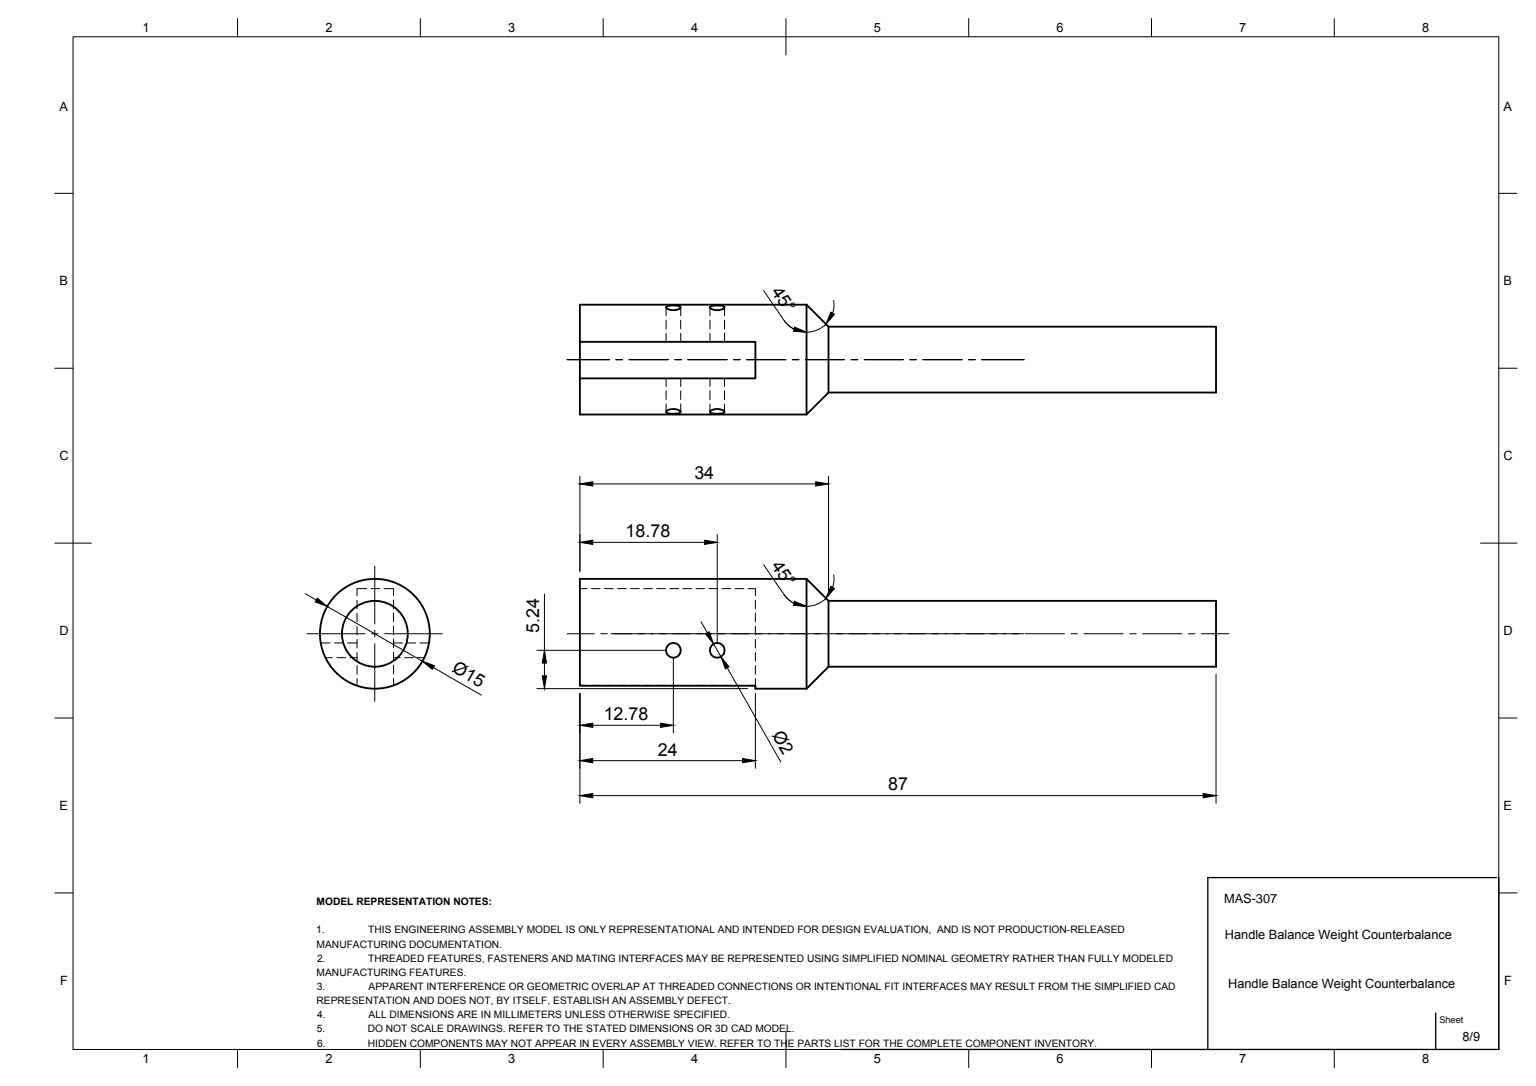
ISO-10303-21;
HEADER;
FILE_DESCRIPTION (('STEP AP214'),
    '1' );
FILE_NAME ('Handle Balance Weight Counterbalance.step',
    '2026-10-06T07:34:29',
    ( '' ),
    ( '' ),
    'SwSTEP 2.0',
    'SolidWorks 2025',
    '' );
FILE_SCHEMA (( 'AUTOMOTIVE_DESIGN' ));
ENDSEC;

DATA;
#24=CARTESIAN_POINT ( 'NONE',  ( -136.1405586187959784, 108.3975249866138597, 0.000000000000000000 ) ) ;
#39=CARTESIAN_POINT ( 'NONE',  ( -152.4086188282879277, 107.2728346664360259, 84.88378295107887084 ) ) ;
#41=CARTESIAN_POINT ( 'NONE',  ( -150.4086188282879277, 107.2728346664360259, 5.000000000000004441 ) ) ;
#42=CONICAL_SURFACE ( 'NONE', #4331, 4.499999999999950262, 0.7853981633974450594 ) ;
#130=EDGE_LOOP ( 'NONE', ( #9688, #11393, #15136, #3970 ) ) ;
#153=CARTESIAN_POINT ( 'NONE',  ( -152.0435700508773209, 108.0561044943065951, -4.829560219627783368 ) ) ;
#169=AXIS2_PLACEMENT_3D ( 'NONE', #9896, #5224, #1587 ) ;
#306=ORIENTED_EDGE ( 'NONE', *, *, #7823, .F. ) ;
#374=EDGE_LOOP ( 'NONE', ( #1367, #9906 ) ) ;
#386=CARTESIAN_POINT ( 'NONE',  ( -217.3071532141029820, 141.4846410501804712, 2.431557144026069928 ) ) ;
#394=ORIENTED_EDGE ( 'NONE', *, *, #3261, .F. ) ;
#397=CARTESIAN_POINT ( 'NONE',  ( -156.1143961258770503, 109.3137364120441077, -4.543781140870884805 ) ) ;
#425=FACE_OUTER_BOUND ( 'NONE', #2124, .T. ) ;
#429=CARTESIAN_POINT ( 'NONE',  ( -166.6414209516114795, 123.5128972754229011, 2.431557144026069928 ) ) ;
#441=AXIS2_PLACEMENT_3D ( 'NONE', #3058, #8986, #15190 ) ;
#451=DIRECTION ( 'NONE',  ( 0.000000000000000000, 0.000000000000000000, -1.000000000000000000 ) ) ;
#472=CARTESIAN_POINT ( 'NONE',  ( -142.6037198098624685, 96.81775716765160666, 0.000000000000000000 ) ) ;
#482=DIRECTION ( 'NONE',  ( -0.4873681696970814659, -0.8731965799097686221, 0.000000000000000000 ) ) ;
#505=EDGE_CURVE ( 'NONE', #2386, #1610, #1044, .T. ) ;
#514=PRESENTATION_STYLE_ASSIGNMENT (( #7896 ) ) ;
#547=CLOSED_SHELL ( 'NONE', ( #13923, #14725, #1343, #11232, #3493, #10653, #12710, #1912, #4244, #2083, #9242, #12419, #15408, #10431, #12199, #12057, #3318, #15550, #7489, #14627 ) ) ;
#588=CARTESIAN_POINT ( 'NONE',  ( -156.1569890673251280, 111.0783851182460893, -4.963902819945231748 ) ) ;
#594=CARTESIAN_POINT ( 'NONE',  ( -150.6118892440573802, 107.8916133795084846, 9.813105602333695998 ) ) ;
#621=ORIENTED_EDGE ( 'NONE', *, *, #1015, .F. ) ;
#638=DIRECTION ( 'NONE',  ( 0.000000000000000000, -0.000000000000000000, -1.000000000000000000 ) ) ;
#663=CARTESIAN_POINT ( 'NONE',  ( -155.8520457446764453, 110.8171731141052163, -4.950117075408069667 ) ) ;
#721=CARTESIAN_POINT ( 'NONE',  ( -155.6477983077465410, 110.1970436846185066, 84.88378295107887084 ) ) ;
#735=CARTESIAN_POINT ( 'NONE',  ( -152.4086188282879277, 107.2728346664360402, -4.548387523817075895 ) ) ;
#744=CARTESIAN_POINT ( 'NONE',  ( -157.1749258454821927, 111.0568882623570062, -4.859112388478813216 ) ) ;
#750=AXIS2_PLACEMENT_3D ( 'NONE', #11545, #7934, #3105 ) ;
#788=EDGE_LOOP ( 'NONE', ( #3520, #15305, #7596, #11160 ) ) ;
#858=VERTEX_POINT ( 'NONE', #6644 ) ;
#882=FACE_OUTER_BOUND ( 'NONE', #8952, .T. ) ;
#907=EDGE_LOOP ( 'NONE', ( #8993, #12549, #11670, #14820 ) ) ;
#909=CARTESIAN_POINT ( 'NONE',  ( -152.2204635237962691, 107.8706385701098185, 9.623760898223435944 ) ) ;
#981=CARTESIAN_POINT ( 'NONE',  ( -156.6477983077465410, 110.1970436846185066, 84.88378295107887084 ) ) ;
#1015=EDGE_CURVE ( 'NONE', #14712, #13022, #15364, .T. ) ;
#1025=EDGE_CURVE ( 'NONE', #9103, #13250, #7487, .T. ) ;
#1036=CARTESIAN_POINT ( 'NONE',  ( -152.2117530991619958, 106.6622082107205216, 9.223488592771907690 ) ) ;
#1044=CIRCLE ( 'NONE', #5333, 7.499999999999999112 ) ;
#1048=LINE ( 'NONE', #6988, #13883 ) ;
#1056=FACE_OUTER_BOUND ( 'NONE', #9716, .T. ) ;
#1084=CARTESIAN_POINT ( 'NONE',  ( -156.6477983077465410, 110.1970436846185066, 5.000000000000004441 ) ) ;
#1086=EDGE_LOOP ( 'NONE', ( #8415, #5150, #14250, #3362 ) ) ;
#1142=CYLINDRICAL_SURFACE ( 'NONE', #13573, 1.000000000000000888 ) ;
#1158=CARTESIAN_POINT ( 'NONE',  ( -157.6477983077465694, 110.0680497146841077, 9.367218745794341217 ) ) ;
#1159=DIRECTION ( 'NONE',  ( 0.000000000000000000, -0.000000000000000000, -1.000000000000000000 ) ) ;
#1177=ORIENTED_EDGE ( 'NONE', *, *, #7018, .T. ) ;
#1191=CARTESIAN_POINT ( 'NONE',  ( -150.9178095878665715, 108.1541761000636086, -4.963902819945232636 ) ) ;
#1200=DIRECTION ( 'NONE',  ( 0.2728218852358202384, -0.9620645606903794889, 8.659560562354905741E-17 ) ) ;
#1234=EDGE_CURVE ( 'NONE', #4804, #2746, #9270, .T. ) ;
#1285=CYLINDRICAL_SURFACE ( 'NONE', #12239, 4.499999999999950262 ) ;
#1315=CARTESIAN_POINT ( 'NONE',  ( -157.5246693090277006, 109.6988848934566647, 9.252772226370421293 ) ) ;
#1333=VERTEX_POINT ( 'NONE', #7170 ) ;
#1337=DIRECTION ( 'NONE',  ( 0.000000000000000000, 0.000000000000000000, -1.000000000000000000 ) ) ;
#1343=ADVANCED_FACE ( 'NONE', ( #11973 ), #5969, .F. ) ;
#1351=CARTESIAN_POINT ( 'NONE',  ( -157.0972765366304316, 120.0943610593438251, 0.000000000000000000 ) ) ;
#1352=CARTESIAN_POINT ( 'NONE',  ( -150.8031737844540601, 108.0798160477858261, -4.962432776364140707 ) ) ;
#1367=ORIENTED_EDGE ( 'NONE', *, *, #6082, .F. ) ;
#1404=ORIENTED_EDGE ( 'NONE', *, *, #8963, .T. ) ;
#1410=ORIENTED_EDGE ( 'NONE', *, *, #1015, .T. ) ;
#1435=CARTESIAN_POINT ( 'NONE',  ( -155.6745145678418680, 109.9335888524736049, -4.794633519332698768 ) ) ;
#1509=CARTESIAN_POINT ( 'NONE',  ( -156.1541198758405358, 111.0769426152140369, 9.827040175762295604 ) ) ;
#1557=CARTESIAN_POINT ( 'NONE',  ( -151.9345376450077367, 108.1333972819248004, 9.722517344254141491 ) ) ;
#1565=VERTEX_POINT ( 'NONE', #12048 ) ;
#1587=DIRECTION ( 'NONE',  ( -1.000000000000000000, 0.000000000000000000, 0.000000000000000000 ) ) ;
#1588=ORIENTED_EDGE ( 'NONE', *, *, #4992, .F. ) ;
#1589=CARTESIAN_POINT ( 'NONE',  ( -143.5695094297736034, 95.08739346018396077, 5.000000000000000000 ) ) ;
#1608=EDGE_CURVE ( 'NONE', #6618, #13250, #10348, .T. ) ;
#1609=DIRECTION ( 'NONE',  ( -0.4873681696970814659, -0.8731965799097686221, 0.000000000000000000 ) ) ;
#1610=VERTEX_POINT ( 'NONE', #472 ) ;
#1630=CARTESIAN_POINT ( 'NONE',  ( -156.8034031652508133, 111.1936819864191506, -4.924812526309167104 ) ) ;
#1655=AXIS2_PLACEMENT_3D ( 'NONE', #1589, #2630, #6426 ) ;
#1665=CARTESIAN_POINT ( 'NONE',  ( -155.6477983077462568, 110.3268634018094758, 9.747367390575373491 ) ) ;
#1672=EDGE_LOOP ( 'NONE', ( #11745, #12944 ) ) ;
#1778=EDGE_CURVE ( 'NONE', #858, #4152, #11112, .T. ) ;
#1784=CARTESIAN_POINT ( 'NONE',  ( -156.5388943062064584, 111.1998600659882896, -4.950241352008077023 ) ) ;
#1788=ORIENTED_EDGE ( 'NONE', *, *, #7310, .T. ) ;
#1792=SURFACE_STYLE_FILL_AREA ( #5434 ) ;
#1850=EDGE_CURVE ( 'NONE', #15505, #12940, #4802, .T. ) ;
#1867=DIRECTION ( 'NONE',  ( -0.8731965799097679559, 0.4873681696970824095, 0.000000000000000000 ) ) ;
#1884=CARTESIAN_POINT ( 'NONE',  ( -157.6477983077465694, 110.1970436846184924, 9.411501811869198875 ) ) ;
#1887=VECTOR ( 'NONE', #7298, 1000.000000000000000 ) ;
#1891=ORIENTED_EDGE ( 'NONE', *, *, #15273, .T. ) ;
#1900=CARTESIAN_POINT ( 'NONE',  ( -156.6477983077465410, 110.1970436846185066, 84.88378295107887084 ) ) ;
#1912=ADVANCED_FACE ( 'NONE', ( #10679, #15472, #4668 ), #13915, .T. ) ;
#1916=FACE_OUTER_BOUND ( 'NONE', #13980, .T. ) ;
#1925=CARTESIAN_POINT ( 'NONE',  ( -150.6072264393035027, 106.6613139020875423, -4.675203989473062371 ) ) ;
#1980=AXIS2_PLACEMENT_3D ( 'NONE', #6052, #11021, #9683 ) ;
#2014=FACE_OUTER_BOUND ( 'NONE', #8148, .T. ) ;
#2016=ORIENTED_EDGE ( 'NONE', *, *, #6082, .T. ) ;
#2066=ADVANCED_BREP_SHAPE_REPRESENTATION ( '', ( #5622, #12337 ), #10297 ) ;
#2070=DIRECTION ( 'NONE',  ( 0.000000000000000000, 0.000000000000000000, -1.000000000000000000 ) ) ;
#2083=ADVANCED_FACE ( 'NONE', ( #3484 ), #13106, .F. ) ;
#2099=DIRECTION ( 'NONE',  ( 0.000000000000000000, 0.000000000000000000, -1.000000000000000000 ) ) ;
#2104=ORIENTED_EDGE ( 'NONE', *, *, #14518, .T. ) ;
#2110=AXIS2_PLACEMENT_3D ( 'NONE', #11190, #2821, #13614 ) ;
#2124=EDGE_LOOP ( 'NONE', ( #15529, #10353, #3293, #4269 ) ) ;
#2136=DIRECTION ( 'NONE',  ( 0.000000000000000000, 0.000000000000000000, -1.000000000000000000 ) ) ;
#2159=VECTOR ( 'NONE', #14026, 1000.000000000000114 ) ;
#2242=CARTESIAN_POINT ( 'NONE',  ( -151.9050178466339105, 106.3942781637374679, -4.320071790863974748 ) ) ;
#2263=DIRECTION ( 'NONE',  ( 1.000000000000000000, 0.000000000000000000, 0.000000000000000000 ) ) ;
#2271=CARTESIAN_POINT ( 'NONE',  ( -156.3659111473432404, 109.2018789623903814, 9.312033302791148159 ) ) ;
#2284=EDGE_CURVE ( 'NONE', #8811, #8894, #6726, .T. ) ;
#2302=CARTESIAN_POINT ( 'NONE',  ( -150.6066609957502180, 106.6619251280432223, 9.538603418629666209 ) ) ;
#2303=DIRECTION ( 'NONE',  ( -0.4873681696970824651, -0.8731965799097680669, 0.000000000000000000 ) ) ;
#2323=CIRCLE ( 'NONE', #11152, 1.000000000000000888 ) ;
#2353=CARTESIAN_POINT ( 'NONE',  ( -171.0277344788851792, 115.6541280562350664, 2.431557144026069928 ) ) ;
#2386=VERTEX_POINT ( 'NONE', #3316 ) ;
#2392=DIRECTION ( 'NONE',  ( -0.8731965799097685110, 0.4873681696970817434, 0.000000000000000000 ) ) ;
#2400=CARTESIAN_POINT ( 'NONE',  ( -151.4086188282879277, 107.2728346664360259, 84.88378295107887084 ) ) ;
#2421=CIRCLE ( 'NONE', #7731, 1.000000000000000888 ) ;
#2428=CARTESIAN_POINT ( 'NONE',  ( -155.6744015425144312, 109.9339595500499343, 9.657855017614867421 ) ) ;
#2434=( NAMED_UNIT ( * ) SI_UNIT ( $, .STERADIAN. ) SOLID_ANGLE_UNIT ( ) );
#2440=DIRECTION ( 'NONE',  ( 0.8731965799097684000, -0.4873681696970815769, -0.000000000000000000 ) ) ;
#2475=DIRECTION ( 'NONE',  ( -1.000000000000000000, 0.000000000000000000, 0.000000000000000000 ) ) ;
#2525=AXIS2_PLACEMENT_3D ( 'NONE', #10287, #638, #6595 ) ;
#2536=ORIENTED_EDGE ( 'NONE', *, *, #2882, .F. ) ;
#2545=EDGE_CURVE ( 'NONE', #858, #12940, #3625, .T. ) ;
#2563=VECTOR ( 'NONE', #14577, 999.9999999999998863 ) ;
#2564=ORIENTED_EDGE ( 'NONE', *, *, #6517, .F. ) ;
#2586=DIRECTION ( 'NONE',  ( 0.000000000000000000, 0.000000000000000000, -1.000000000000000000 ) ) ;
#2590=CARTESIAN_POINT ( 'NONE',  ( -157.1465583139810178, 109.3199373332567603, 9.183240261263447834 ) ) ;
#2597=DIRECTION ( 'NONE',  ( -0.8731965799097685110, 0.4873681696970816324, -0.000000000000000000 ) ) ;
#2598=CARTESIAN_POINT ( 'NONE',  ( -168.8345777152483151, 119.5835126658289909, 2.431557144026069928 ) ) ;
#2618=CARTESIAN_POINT ( 'NONE',  ( -150.5341340129182583, 106.7708477820315665, 9.581378567423383785 ) ) ;
#2630=DIRECTION ( 'NONE',  ( -0.000000000000000000, 0.000000000000000000, 1.000000000000000000 ) ) ;
#2675=LINE ( 'NONE', #14661, #2563 ) ;
#2697=CARTESIAN_POINT ( 'NONE',  ( -152.4086188282879277, 107.2728346664360259, 0.000000000000000000 ) ) ;
#2726=FACE_OUTER_BOUND ( 'NONE', #6526, .T. ) ;
#2746=VERTEX_POINT ( 'NONE', #11432 ) ;
#2802=AXIS2_PLACEMENT_3D ( 'NONE', #14369, #9570, #2303 ) ;
#2821=DIRECTION ( 'NONE',  ( -0.8731965799097685110, 0.4873681696970816324, 0.000000000000000000 ) ) ;
#2865=CARTESIAN_POINT ( 'NONE',  ( -155.8510687235160219, 110.8158223976909369, 9.813105602333695998 ) ) ;
#2868=MECHANICAL_DESIGN_GEOMETRIC_PRESENTATION_REPRESENTATION('',(#11186),#5388);
#2882=EDGE_CURVE ( 'NONE', #11790, #2386, #5470, .T. ) ;
#2906=CARTESIAN_POINT ( 'NONE',  ( -155.6477983077465126, 110.3277548344292995, -4.884442077755424272 ) ) ;
#2933=ORIENTED_EDGE ( 'NONE', *, *, #1234, .F. ) ;
#2962=ORIENTED_EDGE ( 'NONE', *, *, #5310, .T. ) ;
#2981=FACE_BOUND ( 'NONE', #12391, .T. ) ;
#2993=DIRECTION ( 'NONE',  ( -0.000000000000000000, 0.000000000000000000, 1.000000000000000000 ) ) ;
#3058=CARTESIAN_POINT ( 'NONE',  ( -215.1139964504661464, 145.4140256597743814, 2.431557144026069928 ) ) ;
#3083=DIRECTION ( 'NONE',  ( -0.000000000000000000, 0.000000000000000000, 1.000000000000000000 ) ) ;
#3093=VERTEX_POINT ( 'NONE', #14646 ) ;
#3105=DIRECTION ( 'NONE',  ( 0.4873681696970814659, 0.8731965799097686221, 0.000000000000000000 ) ) ;
#3156=ORIENTED_EDGE ( 'NONE', *, *, #5172, .T. ) ;
#3172=ORIENTED_EDGE ( 'NONE', *, *, #5741, .T. ) ;
#3220=FACE_OUTER_BOUND ( 'NONE', #10906, .T. ) ;
#3242=EDGE_LOOP ( 'NONE', ( #3667, #6099, #3351, #12849 ) ) ;
#3261=EDGE_CURVE ( 'NONE', #14091, #858, #3588, .T. ) ;
#3293=ORIENTED_EDGE ( 'NONE', *, *, #12381, .T. ) ;
#3316=CARTESIAN_POINT ( 'NONE',  ( -135.4906327255880569, 109.5619692454514791, 2.431557144026069928 ) ) ;
#3318=ADVANCED_FACE ( 'NONE', ( #1056 ), #15561, .F. ) ;
#3332=EDGE_CURVE ( 'NONE', #13022, #11585, #2421, .T. ) ;
#3335=CARTESIAN_POINT ( 'NONE',  ( -152.4086188282879277, 107.2728346664360259, 9.411501811869209533 ) ) ;
#3351=ORIENTED_EDGE ( 'NONE', *, *, #6517, .T. ) ;
#3359=CARTESIAN_POINT ( 'NONE',  ( -150.4086188282879277, 107.2728346664360259, -4.856732557889654522 ) ) ;
#3362=ORIENTED_EDGE ( 'NONE', *, *, #8963, .F. ) ;
#3443=EDGE_CURVE ( 'NONE', #9203, #8894, #8565, .T. ) ;
#3483=CARTESIAN_POINT ( 'NONE',  ( -150.8759110177108766, 106.3887477331416989, 9.406539233868651095 ) ) ;
#3484=FACE_OUTER_BOUND ( 'NONE', #11779, .T. ) ;
#3493=ADVANCED_FACE ( 'NONE', ( #12334 ), #1285, .T. ) ;
#3506=DIRECTION ( 'NONE',  ( 0.000000000000000000, 0.000000000000000000, -1.000000000000000000 ) ) ;
#3513=ORIENTED_EDGE ( 'NONE', *, *, #4556, .F. ) ;
#3517=CARTESIAN_POINT ( 'NONE',  ( -156.6477983077465410, 110.1970436846185066, 84.88378295107887084 ) ) ;
#3520=ORIENTED_EDGE ( 'NONE', *, *, #3443, .T. ) ;
#3573=VECTOR ( 'NONE', #12281, 1000.000000000000000 ) ;
#3588=LINE ( 'NONE', #8421, #7225 ) ;
#3609=LINE ( 'NONE', #5980, #15367 ) ;
#3613=CARTESIAN_POINT ( 'NONE',  ( -157.6477983077465694, 110.1970436846184924, 9.411501811869198875 ) ) ;
#3625=LINE ( 'NONE', #13241, #13776 ) ;
#3652=CARTESIAN_POINT ( 'NONE',  ( -150.4342454288345721, 107.5345008671435920, -4.906289360893212326 ) ) ;
#3667=ORIENTED_EDGE ( 'NONE', *, *, #10642, .T. ) ;
#3669=DIRECTION ( 'NONE',  ( -0.000000000000000000, -0.000000000000000000, -1.000000000000000000 ) ) ;
#3675=AXIS2_PLACEMENT_3D ( 'NONE', #11931, #9485, #11855 ) ;
#3683=CARTESIAN_POINT ( 'NONE',  ( -150.4086188282879277, 107.2728346664360259, 0.000000000000000000 ) ) ;
#3693=SHAPE_REPRESENTATION_RELATIONSHIP ( 'NONE' , 'NONE' ,  #10258, #2066 ) ;
#3712=CARTESIAN_POINT ( 'NONE',  ( -162.5597267027908401, 124.6703825060609745, 2.431557144026069928 ) ) ;
#3730=CARTESIAN_POINT ( 'NONE',  ( -150.4086188282878425, 107.4035458162468331, -4.884442077755429601 ) ) ;
#3761=AXIS2_PLACEMENT_3D ( 'NONE', #11469, #13584, #14767 ) ;
#3787=AXIS2_PLACEMENT_3D ( 'NONE', #8092, #4432, #13990 ) ;
#3795=ORIENTED_EDGE ( 'NONE', *, *, #12897, .T. ) ;
#3813=FACE_OUTER_BOUND ( 'NONE', #788, .T. ) ;
#3823=CARTESIAN_POINT ( 'NONE',  ( -164.5262273476080850, 106.7842295329139262, 5.000000000000000000 ) ) ;
#3855=CARTESIAN_POINT ( 'NONE',  ( -150.4086188282879277, 107.2728346664360259, 84.88378295107887084 ) ) ;
#3889=FACE_BOUND ( 'NONE', #15005, .T. ) ;
#3930=CARTESIAN_POINT ( 'NONE',  ( -151.5638213263409853, 108.2696846136310711, 9.788006227097797662 ) ) ;
#3932=FACE_OUTER_BOUND ( 'NONE', #4207, .T. ) ;
#3941=PRODUCT_DEFINITION_CONTEXT ( 'detailed design', #11595, 'design' ) ;
#3954=ORIENTED_EDGE ( 'NONE', *, *, #12381, .F. ) ;
#3956=CARTESIAN_POINT ( 'NONE',  ( -157.1737171244663784, 111.0576063001072953, 9.722517344254139715 ) ) ;
#3959=PLANE ( 'NONE',  #3761 ) ;
#3966=CARTESIAN_POINT ( 'NONE',  ( -155.6477983077466263, 110.0646653313681043, -4.828669606760402466 ) ) ;
#3970=ORIENTED_EDGE ( 'NONE', *, *, #2284, .T. ) ;
#4000=CARTESIAN_POINT ( 'NONE',  ( -136.1405586187959784, 108.3975249866138597, 0.000000000000000000 ) ) ;
#4035=DIRECTION ( 'NONE',  ( -0.4873681696970824651, -0.8731965799097680669, 0.000000000000000000 ) ) ;
#4038=ORIENTED_EDGE ( 'NONE', *, *, #4337, .T. ) ;
#4078=EDGE_CURVE ( 'NONE', #5262, #6618, #8618, .T. ) ;
#4086=CARTESIAN_POINT ( 'NONE',  ( -160.1026119161506358, 114.7098309688581708, 2.431557144026069928 ) ) ;
#4107=ORIENTED_EDGE ( 'NONE', *, *, #1778, .T. ) ;
#4127=AXIS2_PLACEMENT_3D ( 'NONE', #5331, #10077, #14948 ) ;
#4148=CARTESIAN_POINT ( 'NONE',  ( -156.9354057470242765, 111.1637277590593982, -4.906715952278847936 ) ) ;
#4152=VERTEX_POINT ( 'NONE', #3712 ) ;
#4156=( NAMED_UNIT ( * ) PLANE_ANGLE_UNIT ( ) SI_UNIT ( $, .RADIAN. ) );
#4173=ORIENTED_EDGE ( 'NONE', *, *, #10294, .F. ) ;
#4207=EDGE_LOOP ( 'NONE', ( #394, #13903, #12494, #9455 ) ) ;
#4230=CARTESIAN_POINT ( 'NONE',  ( -150.9149403963819225, 108.1527335970315420, 9.827040175762299157 ) ) ;
#4233=SURFACE_SIDE_STYLE ('',( #1792 ) ) ;
#4244=ADVANCED_FACE ( 'NONE', ( #13488 ), #12536, .F. ) ;
#4263=FACE_OUTER_BOUND ( 'NONE', #130, .T. ) ;
#4269=ORIENTED_EDGE ( 'NONE', *, *, #12897, .F. ) ;
#4301=EDGE_CURVE ( 'NONE', #13018, #3093, #9168, .T. ) ;
#4305=CARTESIAN_POINT ( 'NONE',  ( -155.7763779997967504, 110.7054720168813731, -4.939346198087217310 ) ) ;
#4331=AXIS2_PLACEMENT_3D ( 'NONE', #2598, #9710, #10898 ) ;
#4337=EDGE_CURVE ( 'NONE', #13018, #5068, #13323, .T. ) ;
#4373=CARTESIAN_POINT ( 'NONE',  ( -212.9208396868292823, 149.3434102693682917, 2.431557144026069928 ) ) ;
#4391=CARTESIAN_POINT ( 'NONE',  ( -166.6414209516114795, 123.5128972754229011, 2.431557144026069928 ) ) ;
#4401=CARTESIAN_POINT ( 'NONE',  ( -155.6477983077465410, 110.1970436846185066, 5.000000000000004441 ) ) ;
#4409=DIRECTION ( 'NONE',  ( -1.000000000000000000, 0.000000000000000000, 0.000000000000000000 ) ) ;
#4432=DIRECTION ( 'NONE',  ( 0.8731965799097690661, -0.4873681696970805222, 0.000000000000000000 ) ) ;
#4435=CARTESIAN_POINT ( 'NONE',  ( -152.4086188282879277, 107.2728346664360259, 84.88378295107887084 ) ) ;
#4440=DIRECTION ( 'NONE',  ( -0.8731965799097684000, 0.4873681696970816879, 0.000000000000000000 ) ) ;
#4488=DIRECTION ( 'NONE',  ( -0.8731965799097685110, 0.4873681696970816324, -0.000000000000000000 ) ) ;
#4503=DIRECTION ( 'NONE',  ( -1.000000000000000000, 0.000000000000000000, 0.000000000000000000 ) ) ;
#4556=EDGE_CURVE ( 'NONE', #8894, #13013, #15523, .T. ) ;
#4568=CARTESIAN_POINT ( 'NONE',  ( 0.000000000000000000, 0.000000000000000000, 0.000000000000000000 ) ) ;
#4579=EDGE_LOOP ( 'NONE', ( #6858, #8658, #5081, #4990, #11443, #4173 ) ) ;
#4634=CARTESIAN_POINT ( 'NONE',  ( -157.0972765366304316, 120.0943610593438251, 0.000000000000000000 ) ) ;
#4667=CARTESIAN_POINT ( 'NONE',  ( -152.2854898295690873, 106.7746758752742124, 9.252772226370428399 ) ) ;
#4668=FACE_BOUND ( 'NONE', #15521, .T. ) ;
#4719=ORIENTED_EDGE ( 'NONE', *, *, #1608, .T. ) ;
#4728=ORIENTED_EDGE ( 'NONE', *, *, #10294, .T. ) ;
#4754=EDGE_CURVE ( 'NONE', #13295, #13013, #13398, .T. ) ;
#4800=CARTESIAN_POINT ( 'NONE',  ( -156.1150904971695752, 109.3129567513242080, 9.406539233868645766 ) ) ;
#4802=CIRCLE ( 'NONE', #14615, 7.499999999999999112 ) ;
#4804=VERTEX_POINT ( 'NONE', #9300 ) ;
#4808=CARTESIAN_POINT ( 'NONE',  ( -157.0972765366304316, 120.0943610593438251, 0.000000000000000000 ) ) ;
#4842=ORIENTED_EDGE ( 'NONE', *, *, #505, .F. ) ;
#4846=ORIENTED_EDGE ( 'NONE', *, *, #505, .T. ) ;
#4854=DIRECTION ( 'NONE',  ( 0.000000000000000000, 0.000000000000000000, -1.000000000000000000 ) ) ;
#4887=ORIENTED_EDGE ( 'NONE', *, *, #13436, .T. ) ;
#4900=ORIENTED_EDGE ( 'NONE', *, *, #5741, .F. ) ;
#4921=FACE_BOUND ( 'NONE', #1672, .T. ) ;
#4924=CARTESIAN_POINT ( 'NONE',  ( -168.8345777152483151, 119.5835126658289909, 2.431557144026069928 ) ) ;
#4950=VECTOR ( 'NONE', #12182, 999.9999999999998863 ) ;
#4952=DIRECTION ( 'NONE',  ( -0.4873681696970814659, -0.8731965799097686221, 0.000000000000000000 ) ) ;
#4982=CARTESIAN_POINT ( 'NONE',  ( -157.6477983077465694, 110.1970436846185066, 84.88378295107887084 ) ) ;
#4990=ORIENTED_EDGE ( 'NONE', *, *, #9412, .T. ) ;
#4992=EDGE_CURVE ( 'NONE', #1333, #14712, #7083, .T. ) ;
#5068=VERTEX_POINT ( 'NONE', #2697 ) ;
#5075=CARTESIAN_POINT ( 'NONE',  ( -152.2908072257909282, 107.7606257468605833, -4.720820933574416678 ) ) ;
#5081=ORIENTED_EDGE ( 'NONE', *, *, #5603, .T. ) ;
#5150=ORIENTED_EDGE ( 'NONE', *, *, #10337, .T. ) ;
#5172=EDGE_CURVE ( 'NONE', #11790, #8811, #14910, .T. ) ;
#5224=DIRECTION ( 'NONE',  ( 0.000000000000000000, 0.000000000000000000, -1.000000000000000000 ) ) ;
#5242=CIRCLE ( 'NONE', #13036, 1.000000000000000888 ) ;
#5262=VERTEX_POINT ( 'NONE', #1884 ) ;
#5289=DIRECTION ( 'NONE',  ( -0.4873681696970815769, -0.8731965799097684000, 0.000000000000000000 ) ) ;
#5299=CARTESIAN_POINT ( 'NONE',  ( -157.6233538794060962, 110.4504304370075829, 9.499964102291375667 ) ) ;
#5310=EDGE_CURVE ( 'NONE', #6421, #4804, #14826, .T. ) ;
#5315=CARTESIAN_POINT ( 'NONE',  ( -155.6477983077465410, 110.1970436846185066, -4.856732557889651858 ) ) ;
#5331=CARTESIAN_POINT ( 'NONE',  ( -151.4086188282879277, 107.2728346664360259, 0.000000000000000000 ) ) ;
#5333=AXIS2_PLACEMENT_3D ( 'NONE', #13680, #8890, #482 ) ;
#5336=DIRECTION ( 'NONE',  ( 0.8731965799097690661, -0.4873681696970805222, 0.000000000000000000 ) ) ;
#5350=DIRECTION ( 'NONE',  ( 0.9620645606903813762, 0.2728218852358138546, 0.000000000000000000 ) ) ;
#5353=( LENGTH_UNIT ( ) NAMED_UNIT ( * ) SI_UNIT ( .MILLI., .METRE. ) );
#5378=VECTOR ( 'NONE', #451, 1000.000000000000000 ) ;
#5384=CARTESIAN_POINT ( 'NONE',  ( -155.6738846654525048, 110.4594052389692962, 9.769471784547329563 ) ) ;
#5388=( GEOMETRIC_REPRESENTATION_CONTEXT ( 3 ) GLOBAL_UNCERTAINTY_ASSIGNED_CONTEXT ( ( #6756 ) ) GLOBAL_UNIT_ASSIGNED_CONTEXT ( ( #5353, #4156, #12680 ) ) REPRESENTATION_CONTEXT ( 'NONE', 'WORKASPACE' ) );
#5432=CARTESIAN_POINT ( 'NONE',  ( -150.8011781171663017, 108.0782419600532620, 9.825479475539731666 ) ) ;
#5434=FILL_AREA_STYLE ('',( #6633 ) ) ;
#5470=CIRCLE ( 'NONE', #6222, 7.499999999999999112 ) ;
#5502=CARTESIAN_POINT ( 'NONE',  ( -155.6477983077465410, 110.1970436846185066, -4.856732557889651858 ) ) ;
#5589=LINE ( 'NONE', #6703, #11121 ) ;
#5601=VECTOR ( 'NONE', #14729, 1000.000000000000000 ) ;
#5603=EDGE_CURVE ( 'NONE', #12940, #9203, #11692, .T. ) ;
#5622=MANIFOLD_SOLID_BREP ( 'Move Face2', #547 ) ;
#5629=DIRECTION ( 'NONE',  ( -0.8731965799097679559, 0.4873681696970824095, 0.000000000000000000 ) ) ;
#5634=CIRCLE ( 'NONE', #13439, 1.000000000000000888 ) ;
#5663=DIRECTION ( 'NONE',  ( 0.8731965799097684000, -0.4873681696970815769, -0.000000000000000000 ) ) ;
#5681=DIRECTION ( 'NONE',  ( 1.000000000000000000, 0.000000000000000000, 0.000000000000000000 ) ) ;
#5701=ORIENTED_EDGE ( 'NONE', *, *, #1234, .T. ) ;
#5706=CARTESIAN_POINT ( 'NONE',  ( -160.1026119161506358, 114.7098309688581708, 2.431557144026069928 ) ) ;
#5713=DIRECTION ( 'NONE',  ( 0.4873681696970831312, 0.8731965799097676229, 0.000000000000000000 ) ) ;
#5739=CARTESIAN_POINT ( 'NONE',  ( -152.3841743999474829, 107.5262214188251164, 9.499964102291382773 ) ) ;
#5741=EDGE_CURVE ( 'NONE', #11585, #13022, #11945, .T. ) ;
#5772=VECTOR ( 'NONE', #11525, 1000.000000000000000 ) ;
#5800=CARTESIAN_POINT ( 'NONE',  ( -150.8752166464184370, 106.3895273938615702, -4.543781140870890134 ) ) ;
#5808=LINE ( 'NONE', #24, #7717 ) ;
#5824=CARTESIAN_POINT ( 'NONE',  ( -136.1405586187959784, 108.3975249866138597, 0.000000000000000000 ) ) ;
#5862=CARTESIAN_POINT ( 'NONE',  ( -151.6579988274852724, 106.2951400763832766, 9.199440363476590221 ) ) ;
#5918=ORIENTED_EDGE ( 'NONE', *, *, #15246, .F. ) ;
#5949=UNCERTAINTY_MEASURE_WITH_UNIT (LENGTH_MEASURE( 1.000000000000000082E-05 ), #13157, 'distance_accuracy_value', 'NONE');
#5954=CARTESIAN_POINT ( 'NONE',  ( -152.4086188282879277, 107.2728346664360402, -4.548387523817075895 ) ) ;
#5968=DIRECTION ( 'NONE',  ( -1.000000000000000000, 0.000000000000000000, 0.000000000000000000 ) ) ;
#5969=CYLINDRICAL_SURFACE ( 'NONE', #12340, 1.000000000000000888 ) ;
#5980=CARTESIAN_POINT ( 'NONE',  ( -136.1405586187959784, 108.3975249866138597, 0.000000000000000000 ) ) ;
#5988=DIRECTION ( 'NONE',  ( 1.000000000000000000, 0.000000000000000000, 0.000000000000000000 ) ) ;
#5994=LINE ( 'NONE', #9629, #6866 ) ;
#6001=VECTOR ( 'NONE', #2597, 999.9999999999998863 ) ;
#6037=CARTESIAN_POINT ( 'NONE',  ( -151.4086188282879277, 107.2728346664360259, 5.000000000000004441 ) ) ;
#6039=DIRECTION ( 'NONE',  ( -1.000000000000000000, 0.000000000000000000, 0.000000000000000000 ) ) ;
#6052=CARTESIAN_POINT ( 'NONE',  ( -151.4086188282879277, 107.2728346664360259, 84.88378295107887084 ) ) ;
#6071=CARTESIAN_POINT ( 'NONE',  ( -157.2622295109954962, 109.3968164531734857, 9.188529295497616545 ) ) ;
#6082=EDGE_CURVE ( 'NONE', #5068, #13018, #8935, .T. ) ;
#6099=ORIENTED_EDGE ( 'NONE', *, *, #12184, .T. ) ;
#6110=CARTESIAN_POINT ( 'NONE',  ( -151.6962262675657200, 108.2395187408769033, -4.906715952278851489 ) ) ;
#6118=DIRECTION ( 'NONE',  ( 0.4873681696970831312, 0.8731965799097676229, 0.000000000000000000 ) ) ;
#6122=CARTESIAN_POINT ( 'NONE',  ( -166.2149879755189659, 118.1214081567377150, 2.431557144026069928 ) ) ;
#6222=AXIS2_PLACEMENT_3D ( 'NONE', #12051, #14257, #4952 ) ;
#6255=VERTEX_POINT ( 'NONE', #4373 ) ;
#6257=PRODUCT_CONTEXT ( 'NONE', #14795, 'mechanical' ) ;
#6264=CARTESIAN_POINT ( 'NONE',  ( -152.4086188282878993, 107.4001535559411167, -4.592095542101958472 ) ) ;
#6275=PRODUCT_DEFINITION_FORMATION_WITH_SPECIFIED_SOURCE ( 'ANY', '', #7916, .NOT_KNOWN. ) ;
#6287=ORIENTED_EDGE ( 'NONE', *, *, #7823, .T. ) ;
#6329=VERTEX_POINT ( 'NONE', #5954 ) ;
#6351=EDGE_LOOP ( 'NONE', ( #9846, #8991 ) ) ;
#6421=VERTEX_POINT ( 'NONE', #14623 ) ;
#6424=CARTESIAN_POINT ( 'NONE',  ( -156.0403575966249434, 111.0024509782357285, 9.825479475539728114 ) ) ;
#6426=DIRECTION ( 'NONE',  ( 1.000000000000000000, 0.000000000000000000, 0.000000000000000000 ) ) ;
#6437=CARTESIAN_POINT ( 'NONE',  ( -156.7587144051361179, 109.1946030148509408, -4.358407942927352785 ) ) ;
#6501=CARTESIAN_POINT ( 'NONE',  ( -157.4596430032548540, 110.7948475882922850, 9.623760898223428839 ) ) ;
#6517=EDGE_CURVE ( 'NONE', #2746, #4804, #9724, .T. ) ;
#6526=EDGE_LOOP ( 'NONE', ( #2016, #15260, #1788, #306 ) ) ;
#6546=CARTESIAN_POINT ( 'NONE',  ( -136.1405586187959784, 108.3975249866138597, 0.000000000000000000 ) ) ;
#6557=AXIS2_PLACEMENT_3D ( 'NONE', #4924, #7228, #12097 ) ;
#6595=DIRECTION ( 'NONE',  ( 1.000000000000000000, 0.000000000000000000, 0.000000000000000000 ) ) ;
#6618=VERTEX_POINT ( 'NONE', #8386 ) ;
#6624=CARTESIAN_POINT ( 'NONE',  ( -156.4041773974485920, 111.1759743691806648, -4.957866620889592291 ) ) ;
#6633=FILL_AREA_STYLE_COLOUR ( '', #6666 ) ;
#6644=CARTESIAN_POINT ( 'NONE',  ( -169.8702492482470632, 111.5724338074144413, 2.431557144026070372 ) ) ;
#6666=COLOUR_RGB ( '', 0.09019608, 0.27058824, 0.51372549) ;
#6686=ORIENTED_EDGE ( 'NONE', *, *, #14018, .T. ) ;
#6703=CARTESIAN_POINT ( 'NONE',  ( -172.2688154150754940, 113.4305367422061579, 5.000000000000000000 ) ) ;
#6712=LINE ( 'NONE', #10178, #2159 ) ;
#6726=LINE ( 'NONE', #11690, #15374 ) ;
#6756=UNCERTAINTY_MEASURE_WITH_UNIT (LENGTH_MEASURE( 1.000000000000000082E-05 ), #5353, 'distance_accuracy_value', 'NONE');
#6761=CARTESIAN_POINT ( 'NONE',  ( -151.1262866895993966, 106.2783261085441495, -4.449251264896262548 ) ) ;
#6765=DIRECTION ( 'NONE',  ( -0.000000000000000000, 0.000000000000000000, 1.000000000000000000 ) ) ;
#6844=CARTESIAN_POINT ( 'NONE',  ( -152.3062201278460748, 106.7562614988853369, -4.377525546821595448 ) ) ;
#6848=FACE_OUTER_BOUND ( 'NONE', #13888, .T. ) ;
#6849=ORIENTED_EDGE ( 'NONE', *, *, #14018, .F. ) ;
#6858=ORIENTED_EDGE ( 'NONE', *, *, #10829, .T. ) ;
#6866=VECTOR ( 'NONE', #7197, 1000.000000000000114 ) ;
#6974=AXIS2_PLACEMENT_3D ( 'NONE', #2400, #4854, #2475 ) ;
#6977=CARTESIAN_POINT ( 'NONE',  ( -152.4086188282879561, 107.1438406965016554, 9.367218745794350099 ) ) ;
#6988=CARTESIAN_POINT ( 'NONE',  ( -219.9064123261074428, 153.2423556269449421, 2.431557144026069928 ) ) ;
#7018=EDGE_CURVE ( 'NONE', #13295, #1610, #3609, .T. ) ;
#7021=EDGE_CURVE ( 'NONE', #1333, #11585, #15589, .T. ) ;
#7031=ORIENTED_EDGE ( 'NONE', *, *, #4301, .F. ) ;
#7058=AXIS2_PLACEMENT_3D ( 'NONE', #14307, #3506, #6039 ) ;
#7077=CARTESIAN_POINT ( 'NONE',  ( -152.0205871941159614, 106.4705699334293598, -4.325135862343421955 ) ) ;
#7083=B_SPLINE_CURVE_WITH_KNOTS ( 'NONE', 3,
 ( #3335, #6977, #11862, #4667, #1036, #11939, #12954, #5862, #9494, #14290, #3483, #2302, #2618, #7597, #9652, #13338 ),
 .UNSPECIFIED., .F., .F.,
 ( 4, 2, 2, 2, 2, 2, 2, 4 ),
 ( 0.000000000000000000, 0.0004036473355434109611, 0.0008072946710868219222, 0.001210942006630233046, 0.001614589342173643844, 0.002421884013260385427, 0.002825531348803770638, 0.003229178684347154982 ),
 .UNSPECIFIED. ) ;
#7154=DIRECTION ( 'NONE',  ( 0.000000000000000000, -0.000000000000000000, -1.000000000000000000 ) ) ;
#7170=CARTESIAN_POINT ( 'NONE',  ( -152.4086188282879277, 107.2728346664360259, 9.411501811869209533 ) ) ;
#7197=DIRECTION ( 'NONE',  ( 0.8731965799097684000, -0.4873681696970815769, -0.000000000000000000 ) ) ;
#7225=VECTOR ( 'NONE', #1200, 1000.000000000000114 ) ;
#7228=DIRECTION ( 'NONE',  ( -0.8731965799097685110, 0.4873681696970816324, 0.000000000000000000 ) ) ;
#7260=CARTESIAN_POINT ( 'NONE',  ( -155.6477983077462852, 110.0653742669871917, 9.691934182417337951 ) ) ;
#7293=CIRCLE ( 'NONE', #441, 4.499999999999950262 ) ;
#7298=DIRECTION ( 'NONE',  ( 0.000000000000000000, 0.000000000000000000, -1.000000000000000000 ) ) ;
#7310=EDGE_CURVE ( 'NONE', #3093, #6329, #11205, .T. ) ;
#7381=CARTESIAN_POINT ( 'NONE',  ( -152.3848650261365663, 107.5241111436813242, -4.636096941365081214 ) ) ;
#7390=DIRECTION ( 'NONE',  ( 0.8731965799097684000, -0.4873681696970816324, -0.000000000000000000 ) ) ;
#7395=DIRECTION ( 'NONE',  ( 0.8731965799097690661, -0.4873681696970805222, 0.000000000000000000 ) ) ;
#7459=CARTESIAN_POINT ( 'NONE',  ( -156.3654661690580667, 109.2025351267266586, -4.449251264896256330 ) ) ;
#7460=CARTESIAN_POINT ( 'NONE',  ( -222.0995690897442785, 149.3129710173510318, 2.431557144026069928 ) ) ;
#7487=LINE ( 'NONE', #12212, #5601 ) ;
#7488=ORIENTED_EDGE ( 'NONE', *, *, #14518, .F. ) ;
#7489=ADVANCED_FACE ( 'NONE', ( #8568 ), #15491, .F. ) ;
#7530=CARTESIAN_POINT ( 'NONE',  ( -151.9357463660236078, 108.1326792441745255, -4.859112388478815880 ) ) ;
#7570=PLANE ( 'NONE',  #14379 ) ;
#7596=ORIENTED_EDGE ( 'NONE', *, *, #5172, .F. ) ;
#7597=CARTESIAN_POINT ( 'NONE',  ( -150.4352220630557895, 107.0097505318674393, 9.657855017614867421 ) ) ;
#7621=CARTESIAN_POINT ( 'NONE',  ( -155.7734221399892363, 109.6948923088348806, -4.718200141660416236 ) ) ;
#7649=CARTESIAN_POINT ( 'NONE',  ( -157.5299867052495699, 110.6848347650430782, -4.720820933574413125 ) ) ;
#7687=CARTESIAN_POINT ( 'NONE',  ( -157.2824335677085799, 110.9804333728871057, 9.692725945294363044 ) ) ;
#7717=VECTOR ( 'NONE', #3669, 1000.000000000000000 ) ;
#7731=AXIS2_PLACEMENT_3D ( 'NONE', #6037, #7154, #10699 ) ;
#7813=ORIENTED_EDGE ( 'NONE', *, *, #3332, .T. ) ;
#7823=EDGE_CURVE ( 'NONE', #5068, #6329, #10451, .T. ) ;
#7829=ORIENTED_EDGE ( 'NONE', *, *, #4992, .T. ) ;
#7838=CARTESIAN_POINT ( 'NONE',  ( -157.6477983077465694, 110.1970436846185066, 84.88378295107887084 ) ) ;
#7847=FACE_OUTER_BOUND ( 'NONE', #3242, .T. ) ;
#7889=CARTESIAN_POINT ( 'NONE',  ( -157.4608918519057568, 110.7933268109660787, -4.760088435541717011 ) ) ;
#7896=SURFACE_STYLE_USAGE ( .BOTH. , #4233 ) ;
#7911=CARTESIAN_POINT ( 'NONE',  ( -151.4086188282879277, 107.2728346664360259, 0.000000000000000000 ) ) ;
#7916=PRODUCT ( 'Handle Balance Weight Counterbalance', 'Handle Balance Weight Counterbalance', '', ( #6257 ) ) ;
#7926=B_SPLINE_CURVE_WITH_KNOTS ( 'NONE', 3,
 ( #3613, #1158, #12135, #1315, #10805, #6071, #2590, #9537, #10964, #2271, #4800, #8448, #13228, #2428, #7260, #8518 ),
 .UNSPECIFIED., .F., .F.,
 ( 4, 2, 2, 2, 2, 2, 2, 4 ),
 ( 1.430489624538199204E-17, 0.0004036473355434303683, 0.0008072946710868464252, 0.001210942006630262536, 0.001614589342173678539, 0.002421884013260430530, 0.002825531348803793190, 0.003229178684347155416 ),
 .UNSPECIFIED. ) ;
#7934=DIRECTION ( 'NONE',  ( 0.8731965799097685110, -0.4873681696970816324, -0.000000000000000000 ) ) ;
#7946=ORIENTED_EDGE ( 'NONE', *, *, #7021, .T. ) ;
#7954=CARTESIAN_POINT ( 'NONE',  ( -150.4086188282879277, 107.1404563131855809, -4.828669606760403354 ) ) ;
#8003=CARTESIAN_POINT ( 'NONE',  ( -163.5604377276969217, 108.5145932403815721, 0.000000000000000000 ) ) ;
#8078=EDGE_LOOP ( 'NONE', ( #11298, #6849 ) ) ;
#8092=CARTESIAN_POINT ( 'NONE',  ( -166.2149879755189659, 118.1214081567377150, 2.431557144026069928 ) ) ;
#8143=DIRECTION ( 'NONE',  ( -1.000000000000000000, 0.000000000000000000, 0.000000000000000000 ) ) ;
#8147=DIRECTION ( 'NONE',  ( 0.000000000000000000, 0.000000000000000000, 1.000000000000000000 ) ) ;
#8148=EDGE_LOOP ( 'NONE', ( #12851, #13554, #2962, #5701 ) ) ;
#8196=CARTESIAN_POINT ( 'NONE',  ( -150.4353350883832832, 107.0093798342911242, -4.794633519332702321 ) ) ;
#8238=B_SPLINE_CURVE_WITH_KNOTS ( 'NONE', 3,
 ( #11430, #13544, #8752, #9943, #594, #5432, #4230, #9069, #14734, #3930, #12372, #1557, #12834, #909, #11512, #5739, #13950, #9223 ),
 .UNSPECIFIED., .F., .F.,
 ( 4, 2, 2, 2, 2, 2, 2, 2, 4 ),
 ( 0.003229178684347154982, 0.003627155556181206521, 0.004025132428015258494, 0.004423109299849310033, 0.004821086171683361572, 0.005219063043517413111, 0.005617039915351465518, 0.006015016787185517057, 0.006412993659019568596 ),
 .UNSPECIFIED. ) ;
#8280=EDGE_LOOP ( 'NONE', ( #11760, #6686, #11839, #4719 ) ) ;
#8380=EDGE_CURVE ( 'NONE', #8424, #4152, #12601, .T. ) ;
#8384=EDGE_CURVE ( 'NONE', #14712, #1333, #8238, .T. ) ;
#8386=CARTESIAN_POINT ( 'NONE',  ( -157.6477983077465694, 110.1970436846185066, 5.000000000000004441 ) ) ;
#8396=FACE_BOUND ( 'NONE', #15020, .T. ) ;
#8407=VECTOR ( 'NONE', #2070, 1000.000000000000000 ) ;
#8411=CYLINDRICAL_SURFACE ( 'NONE', #15242, 4.499999999999950262 ) ;
#8415=ORIENTED_EDGE ( 'NONE', *, *, #9015, .F. ) ;
#8419=ORIENTED_EDGE ( 'NONE', *, *, #3261, .T. ) ;
#8421=CARTESIAN_POINT ( 'NONE',  ( -171.0277344788851792, 115.6541280562350806, 2.431557144026069928 ) ) ;
#8423=AXIS2_PLACEMENT_3D ( 'NONE', #11824, #14256, #2263 ) ;
#8424=VERTEX_POINT ( 'NONE', #4391 ) ;
#8448=CARTESIAN_POINT ( 'NONE',  ( -155.8458404752088313, 109.5861341462257172, 9.538603418629666209 ) ) ;
#8450=CARTESIAN_POINT ( 'NONE',  ( -157.0972765366304316, 120.0943610593438251, 5.000000000000000000 ) ) ;
#8487=DIRECTION ( 'NONE',  ( 0.8731965799097685110, -0.4873681696970816879, -0.000000000000000000 ) ) ;
#8488=CARTESIAN_POINT ( 'NONE',  ( -151.2997148267479020, 108.2756510478057947, -4.950241352008081464 ) ) ;
#8518=CARTESIAN_POINT ( 'NONE',  ( -155.6477983077465410, 110.1970436846185066, 9.719846845941789937 ) ) ;
#8552=VECTOR ( 'NONE', #12065, 1000.000000000000000 ) ;
#8565=LINE ( 'NONE', #3823, #4950 ) ;
#8568=FACE_OUTER_BOUND ( 'NONE', #9007, .T. ) ;
#8618=LINE ( 'NONE', #4982, #8798 ) ;
#8642=CARTESIAN_POINT ( 'NONE',  ( -157.5453996073046881, 109.6804705170678034, -4.377525546821591007 ) ) ;
#8658=ORIENTED_EDGE ( 'NONE', *, *, #2545, .T. ) ;
#8682=CIRCLE ( 'NONE', #2110, 4.499999999999950262 ) ;
#8709=CARTESIAN_POINT ( 'NONE',  ( -155.6477983077465410, 110.1970436846185066, 9.719846845941789937 ) ) ;
#8752=CARTESIAN_POINT ( 'NONE',  ( -150.4347051859938915, 107.5351962207867871, 9.769471784547334892 ) ) ;
#8768=CARTESIAN_POINT ( 'NONE',  ( -139.1458939983161827, 103.0129948961282054, 2.431557144026069928 ) ) ;
#8781=CARTESIAN_POINT ( 'NONE',  ( -157.5298637219052296, 110.6847670947880573, 9.583914075210627104 ) ) ;
#8795=CARTESIAN_POINT ( 'NONE',  ( -157.2597666735746031, 109.3947789516118405, -4.325135862343416626 ) ) ;
#8798=VECTOR ( 'NONE', #1337, 1000.000000000000000 ) ;
#8811=VERTEX_POINT ( 'NONE', #10259 ) ;
#8812=AXIS2_PLACEMENT_3D ( 'NONE', #8768, #12389, #5289 ) ;
#8830=ORIENTED_EDGE ( 'NONE', *, *, #11927, .T. ) ;
#8881=CARTESIAN_POINT ( 'NONE',  ( -157.6477983077465410, 109.9391580343927473, -4.459856507254698954 ) ) ;
#8890=DIRECTION ( 'NONE',  ( -0.8731965799097685110, 0.4873681696970816324, 0.000000000000000000 ) ) ;
#8894=VERTEX_POINT ( 'NONE', #8450 ) ;
#8935=CIRCLE ( 'NONE', #4127, 1.000000000000000888 ) ;
#8944=PRODUCT_DEFINITION ( 'UNKNOWN', '', #6275, #3941 ) ;
#8952=EDGE_LOOP ( 'NONE', ( #13056, #7488, #1404, #4887 ) ) ;
#8963=EDGE_CURVE ( 'NONE', #6255, #8424, #1048, .T. ) ;
#8986=DIRECTION ( 'NONE',  ( -0.8731965799097685110, 0.4873681696970817434, 0.000000000000000000 ) ) ;
#8991=ORIENTED_EDGE ( 'NONE', *, *, #7310, .F. ) ;
#8993=ORIENTED_EDGE ( 'NONE', *, *, #11447, .T. ) ;
#8998=CARTESIAN_POINT ( 'NONE',  ( -163.7578731888787331, 108.1608566195349113, 2.431557144026070372 ) ) ;
#9007=EDGE_LOOP ( 'NONE', ( #7031, #4038, #6287, #1891 ) ) ;
#9015=EDGE_CURVE ( 'NONE', #12471, #6255, #12109, .T. ) ;
#9021=CYLINDRICAL_SURFACE ( 'NONE', #169, 1.000000000000000888 ) ;
#9069=CARTESIAN_POINT ( 'NONE',  ( -151.1638989062950031, 108.2516363225298619, 9.821053999514628430 ) ) ;
#9077=AXIS2_PLACEMENT_3D ( 'NONE', #1900, #2136, #4503 ) ;
#9103=VERTEX_POINT ( 'NONE', #11776 ) ;
#9147=CARTESIAN_POINT ( 'NONE',  ( -155.6734249082932422, 110.4587098853260585, -4.906289360893208773 ) ) ;
#9168=LINE ( 'NONE', #14038, #5772 ) ;
#9203=VERTEX_POINT ( 'NONE', #10090 ) ;
#9223=CARTESIAN_POINT ( 'NONE',  ( -152.4086188282879277, 107.2728346664360259, 9.411501811869209533 ) ) ;
#9233=DIRECTION ( 'NONE',  ( 0.000000000000000000, 0.000000000000000000, -1.000000000000000000 ) ) ;
#9242=ADVANCED_FACE ( 'NONE', ( #2981, #11196, #425 ), #7570, .F. ) ;
#9270=B_SPLINE_CURVE_WITH_KNOTS ( 'NONE', 3,
 ( #12595, #14957, #13703, #7649, #7889, #12441, #744, #4148, #1630, #1784, #6624, #588, #15034, #663, #4305, #9147, #2906, #5502 ),
 .UNSPECIFIED., .F., .F.,
 ( 4, 2, 2, 2, 2, 2, 2, 2, 4 ),
 ( 1.482148387583608474E-17, 0.0003981710496980508571, 0.0007963420993960869691, 0.001194513149094122810, 0.001592684198792158976, 0.001990855248490195142, 0.002389026298188230875, 0.002787197347886267041, 0.003185368397584303207 ),
 .UNSPECIFIED. ) ;
#9273=DIRECTION ( 'NONE',  ( -0.4873681696970816879, -0.8731965799097684000, 0.000000000000000000 ) ) ;
#9300=CARTESIAN_POINT ( 'NONE',  ( -157.6477983077465694, 110.1970436846185208, -4.548387523817069678 ) ) ;
#9324=CIRCLE ( 'NONE', #6557, 4.499999999999950262 ) ;
#9412=EDGE_CURVE ( 'NONE', #9203, #11790, #5589, .T. ) ;
#9440=CARTESIAN_POINT ( 'NONE',  ( -151.6539382783454926, 106.2940129864185366, -4.336802791931510193 ) ) ;
#9455=ORIENTED_EDGE ( 'NONE', *, *, #1778, .F. ) ;
#9485=DIRECTION ( 'NONE',  ( 0.8731965799097685110, -0.4873681696970816324, -0.000000000000000000 ) ) ;
#9494=CARTESIAN_POINT ( 'NONE',  ( -151.5230023344471704, 106.2706521918282903, 9.220837571243215791 ) ) ;
#9537=CARTESIAN_POINT ( 'NONE',  ( -156.8971783069440278, 109.2193490945657430, 9.199440363476590221 ) ) ;
#9550=PRODUCT_DEFINITION_SHAPE ( 'NONE', 'NONE',  #8944 ) ;
#9570=DIRECTION ( 'NONE',  ( -0.8731965799097680669, 0.4873681696970824651, 0.000000000000000000 ) ) ;
#9580=CARTESIAN_POINT ( 'NONE',  ( -150.6128662652177752, 107.8929640959227356, -4.950117075408072331 ) ) ;
#9629=CARTESIAN_POINT ( 'NONE',  ( -165.1793164425202178, 126.1324870151522504, 2.431557144026069928 ) ) ;
#9652=CARTESIAN_POINT ( 'NONE',  ( -150.4086188282876719, 107.1411652488047253, 9.691934182417341503 ) ) ;
#9660=DIRECTION ( 'NONE',  ( 0.8731965799097684000, -0.4873681696970816324, -0.000000000000000000 ) ) ;
#9680=CARTESIAN_POINT ( 'NONE',  ( -142.5801316981433615, 96.86001897250537240, 5.000000000000000000 ) ) ;
#9683=DIRECTION ( 'NONE',  ( -1.000000000000000000, 0.000000000000000000, 0.000000000000000000 ) ) ;
#9688=ORIENTED_EDGE ( 'NONE', *, *, #4556, .T. ) ;
#9710=DIRECTION ( 'NONE',  ( 0.8731965799097690661, -0.4873681696970805222, 0.000000000000000000 ) ) ;
#9716=EDGE_LOOP ( 'NONE', ( #621, #10955, #7946, #3172 ) ) ;
#9724=B_SPLINE_CURVE_WITH_KNOTS ( 'NONE', 3,
 ( #5315, #3966, #1435, #7621, #12414, #397, #7459, #6437, #14852, #13440, #8795, #8642, #8881, #13672 ),
 .UNSPECIFIED., .F., .F.,
 ( 4, 2, 2, 2, 2, 2, 4 ),
 ( 0.003185368397584303207, 0.003588618066394591230, 0.003991867735204879253, 0.004798367072825484789, 0.005201616741635828323, 0.005604866410446171857, 0.006411365748066773056 ),
 .UNSPECIFIED. ) ;
#9846=ORIENTED_EDGE ( 'NONE', *, *, #15273, .F. ) ;
#9896=CARTESIAN_POINT ( 'NONE',  ( -156.6477983077465410, 110.1970436846185066, 84.88378295107887084 ) ) ;
#9906=ORIENTED_EDGE ( 'NONE', *, *, #4337, .F. ) ;
#9940=DIRECTION ( 'NONE',  ( 0.000000000000000000, 0.000000000000000000, -1.000000000000000000 ) ) ;
#9943=CARTESIAN_POINT ( 'NONE',  ( -150.5358285740960014, 107.7783824288041217, 9.802099390037296800 ) ) ;
#10077=DIRECTION ( 'NONE',  ( -0.000000000000000000, 0.000000000000000000, 1.000000000000000000 ) ) ;
#10090=CARTESIAN_POINT ( 'NONE',  ( -163.5368496159778147, 108.5568550452353378, 5.000000000000000000 ) ) ;
#10132=ORIENTED_EDGE ( 'NONE', *, *, #2545, .F. ) ;
#10178=CARTESIAN_POINT ( 'NONE',  ( -172.2924035267946294, 113.3882749373523922, 0.000000000000000000 ) ) ;
#10205=CARTESIAN_POINT ( 'NONE',  ( -155.7750080535546147, 110.7025914469866308, 9.802099390037289695 ) ) ;
#10223=PLANE ( 'NONE',  #14238 ) ;
#10258=SHAPE_REPRESENTATION ( 'Handle Balance Weight Counterbalance', ( #12337 ), #10297 ) ;
#10259=CARTESIAN_POINT ( 'NONE',  ( -136.1405586187959784, 108.3975249866138739, 5.000000000000000000 ) ) ;
#10287=CARTESIAN_POINT ( 'NONE',  ( -156.6477983077465410, 110.1970436846185066, 5.000000000000004441 ) ) ;
#10294=EDGE_CURVE ( 'NONE', #4152, #2386, #5994, .T. ) ;
#10297=( GEOMETRIC_REPRESENTATION_CONTEXT ( 3 ) GLOBAL_UNCERTAINTY_ASSIGNED_CONTEXT ( ( #5949 ) ) GLOBAL_UNIT_ASSIGNED_CONTEXT ( ( #13157, #14497, #2434 ) ) REPRESENTATION_CONTEXT ( 'NONE', 'WORKASPACE' ) );
#10314=CARTESIAN_POINT ( 'NONE',  ( -168.8345777152483151, 119.5835126658289909, 2.431557144026069928 ) ) ;
#10335=CYLINDRICAL_SURFACE ( 'NONE', #10457, 1.000000000000000888 ) ;
#10337=EDGE_CURVE ( 'NONE', #12471, #14091, #2675, .T. ) ;
#10348=CIRCLE ( 'NONE', #2525, 1.000000000000000888 ) ;
#10353=ORIENTED_EDGE ( 'NONE', *, *, #4754, .T. ) ;
#10431=ADVANCED_FACE ( 'NONE', ( #3932 ), #42, .T. ) ;
#10451=LINE ( 'NONE', #4435, #8407 ) ;
#10457=AXIS2_PLACEMENT_3D ( 'NONE', #11679, #9233, #8143 ) ;
#10477=DIRECTION ( 'NONE',  ( -1.000000000000000000, 0.000000000000000000, 0.000000000000000000 ) ) ;
#10512=FACE_OUTER_BOUND ( 'NONE', #8280, .T. ) ;
#10539=B_SPLINE_CURVE_WITH_KNOTS ( 'NONE', 3,
 ( #12022, #6264, #7381, #5075, #14691, #153, #7530, #6110, #14533, #8488, #12327, #1191, #1352, #9580, #13270, #3652, #3730, #11003 ),
 .UNSPECIFIED., .F., .F.,
 ( 4, 2, 2, 2, 2, 2, 2, 2, 4 ),
 ( 1.453963218420191702E-17, 0.0003981710496980498271, 0.0007963420993960851259, 0.001194513149094120425, 0.001592684198792155724, 0.001990855248490191239, 0.002389026298188226538, 0.002787197347886261837, 0.003185368397584297136 ),
 .UNSPECIFIED. ) ;
#10642=EDGE_CURVE ( 'NONE', #6421, #1565, #2323, .T. ) ;
#10653=ADVANCED_FACE ( 'NONE', ( #6848 ), #12896, .T. ) ;
#10679=FACE_OUTER_BOUND ( 'NONE', #12027, .T. ) ;
#10699=DIRECTION ( 'NONE',  ( 1.000000000000000000, 0.000000000000000000, 0.000000000000000000 ) ) ;
#10800=DIRECTION ( 'NONE',  ( -0.4873681696970824651, -0.8731965799097680669, 0.000000000000000000 ) ) ;
#10805=CARTESIAN_POINT ( 'NONE',  ( -157.4509325786206091, 109.5864172289029881, 9.223488592771900585 ) ) ;
#10829=EDGE_CURVE ( 'NONE', #4152, #858, #10844, .T. ) ;
#10844=CIRCLE ( 'NONE', #12090, 7.499999999999999112 ) ;
#10898=DIRECTION ( 'NONE',  ( 0.4873681696970831312, 0.8731965799097676229, 0.000000000000000000 ) ) ;
#10906=EDGE_LOOP ( 'NONE', ( #7829, #1410, #7813, #12179 ) ) ;
#10955=ORIENTED_EDGE ( 'NONE', *, *, #8384, .T. ) ;
#10964=CARTESIAN_POINT ( 'NONE',  ( -156.7621818139058405, 109.1948612100107994, 9.220837571243208686 ) ) ;
#11000=ORIENTED_EDGE ( 'NONE', *, *, #10829, .F. ) ;
#11003=CARTESIAN_POINT ( 'NONE',  ( -150.4086188282879277, 107.2728346664360259, -4.856732557889654522 ) ) ;
#11005=ORIENTED_EDGE ( 'NONE', *, *, #1850, .T. ) ;
#11021=DIRECTION ( 'NONE',  ( 0.000000000000000000, 0.000000000000000000, -1.000000000000000000 ) ) ;
#11101=CYLINDRICAL_SURFACE ( 'NONE', #1980, 1.000000000000000888 ) ;
#11112=CIRCLE ( 'NONE', #3787, 7.499999999999999112 ) ;
#11121=VECTOR ( 'NONE', #5663, 1000.000000000000114 ) ;
#11152=AXIS2_PLACEMENT_3D ( 'NONE', #12665, #6765, #12822 ) ;
#11160=ORIENTED_EDGE ( 'NONE', *, *, #9412, .F. ) ;
#11186=STYLED_ITEM ( 'NONE', ( #514 ), #5622 ) ;
#11190=CARTESIAN_POINT ( 'NONE',  ( -168.8345777152483151, 119.5835126658289909, 2.431557144026069928 ) ) ;
#11196=FACE_BOUND ( 'NONE', #374, .T. ) ;
#11205=B_SPLINE_CURVE_WITH_KNOTS ( 'NONE', 3,
 ( #3359, #7954, #8196, #12974, #1925, #5800, #6761, #15414, #9440, #2242, #7077, #6844, #11884, #735 ),
 .UNSPECIFIED., .F., .F.,
 ( 4, 2, 2, 2, 2, 2, 4 ),
 ( 0.003185368397584297136, 0.003588618066394599470, 0.003991867735204901804, 0.004798367072825479585, 0.005201616741635807506, 0.005604866410446135427, 0.006411365748066763515 ),
 .UNSPECIFIED. ) ;
#11232=ADVANCED_FACE ( 'NONE', ( #3220 ), #10335, .F. ) ;
#11298=ORIENTED_EDGE ( 'NONE', *, *, #11447, .F. ) ;
#11393=ORIENTED_EDGE ( 'NONE', *, *, #4754, .F. ) ;
#11430=CARTESIAN_POINT ( 'NONE',  ( -150.4086188282879277, 107.2728346664360259, 9.719846845941791713 ) ) ;
#11432=CARTESIAN_POINT ( 'NONE',  ( -155.6477983077465410, 110.1970436846185066, -4.856732557889651858 ) ) ;
#11437=AXIS2_PLACEMENT_3D ( 'NONE', #4086, #1867, #12606 ) ;
#11438=CARTESIAN_POINT ( 'NONE',  ( -156.6477983077465410, 110.1970436846185066, 0.000000000000000000 ) ) ;
#11443=ORIENTED_EDGE ( 'NONE', *, *, #2882, .T. ) ;
#11447=EDGE_CURVE ( 'NONE', #5262, #9103, #7926, .T. ) ;
#11469=CARTESIAN_POINT ( 'NONE',  ( -136.1405586187959784, 108.3975249866138597, 0.000000000000000000 ) ) ;
#11512=CARTESIAN_POINT ( 'NONE',  ( -152.2906842424466163, 107.7605580766055766, 9.583914075210632433 ) ) ;
#11525=DIRECTION ( 'NONE',  ( 0.000000000000000000, 0.000000000000000000, -1.000000000000000000 ) ) ;
#11545=CARTESIAN_POINT ( 'NONE',  ( -168.8345777152483151, 119.5835126658289909, 2.431557144026069928 ) ) ;
#11557=LINE ( 'NONE', #721, #1887 ) ;
#11572=DIRECTION ( 'NONE',  ( 0.4873681696970831312, 0.8731965799097676229, 0.000000000000000000 ) ) ;
#11585=VERTEX_POINT ( 'NONE', #12513 ) ;
#11595=APPLICATION_CONTEXT ( 'automotive_design' ) ;
#11615=AXIS2_PLACEMENT_3D ( 'NONE', #14151, #2392, #11792 ) ;
#11670=ORIENTED_EDGE ( 'NONE', *, *, #14145, .T. ) ;
#11679=CARTESIAN_POINT ( 'NONE',  ( -151.4086188282879277, 107.2728346664360259, 84.88378295107887084 ) ) ;
#11690=CARTESIAN_POINT ( 'NONE',  ( -136.1405586187959784, 108.3975249866138597, 5.000000000000000000 ) ) ;
#11692=CIRCLE ( 'NONE', #11437, 7.499999999999999112 ) ;
#11696=B_SPLINE_CURVE_WITH_KNOTS ( 'NONE', 3,
 ( #8709, #1665, #5384, #10205, #2865, #6424, #1509, #13501, #14763, #13738, #14995, #3956, #7687, #6501, #8781, #5299, #14836, #13660 ),
 .UNSPECIFIED., .F., .F.,
 ( 4, 2, 2, 2, 2, 2, 2, 2, 4 ),
 ( 0.003229178684347155416, 0.003627155556181209124, 0.004025132428015262831, 0.004423109299849316105, 0.004821086171683369379, 0.005219063043517423520, 0.005617039915351476793, 0.006015016787185530067, 0.006412993659019584208 ),
 .UNSPECIFIED. ) ;
#11719=CARTESIAN_POINT ( 'NONE',  ( -215.1139964504661464, 145.4140256597743814, 2.431557144026069928 ) ) ;
#11745=ORIENTED_EDGE ( 'NONE', *, *, #1608, .F. ) ;
#11759=ORIENTED_EDGE ( 'NONE', *, *, #3443, .F. ) ;
#11760=ORIENTED_EDGE ( 'NONE', *, *, #1025, .F. ) ;
#11775=CYLINDRICAL_SURFACE ( 'NONE', #3675, 7.499999999999999112 ) ;
#11776=CARTESIAN_POINT ( 'NONE',  ( -155.6477983077465410, 110.1970436846185066, 9.719846845941789937 ) ) ;
#11779=EDGE_LOOP ( 'NONE', ( #3954, #3513, #11759, #14782, #14778 ) ) ;
#11790=VERTEX_POINT ( 'NONE', #9680 ) ;
#11792=DIRECTION ( 'NONE',  ( -0.4873681696970831312, -0.8731965799097676229, 0.000000000000000000 ) ) ;
#11824=CARTESIAN_POINT ( 'NONE',  ( -151.4086188282879277, 107.2728346664360259, 5.000000000000004441 ) ) ;
#11839=ORIENTED_EDGE ( 'NONE', *, *, #4078, .T. ) ;
#11854=ORIENTED_EDGE ( 'NONE', *, *, #3332, .F. ) ;
#11855=DIRECTION ( 'NONE',  ( 0.4873681696970814659, 0.8731965799097686221, 0.000000000000000000 ) ) ;
#11862=CARTESIAN_POINT ( 'NONE',  ( -152.3840324909117214, 107.0166450474691260, 9.325089004845759533 ) ) ;
#11884=CARTESIAN_POINT ( 'NONE',  ( -152.4086188282879277, 107.0149490162102808, -4.459856507254708724 ) ) ;
#11927=EDGE_CURVE ( 'NONE', #8811, #13295, #5808, .T. ) ;
#11931=CARTESIAN_POINT ( 'NONE',  ( -168.8345777152483151, 119.5835126658289909, 2.431557144026069928 ) ) ;
#11939=CARTESIAN_POINT ( 'NONE',  ( -152.0230500315369397, 106.4726074349910760, 9.188529295497623650 ) ) ;
#11945=CIRCLE ( 'NONE', #8423, 1.000000000000000888 ) ;
#11973=FACE_OUTER_BOUND ( 'NONE', #907, .T. ) ;
#12022=CARTESIAN_POINT ( 'NONE',  ( -152.4086188282879277, 107.2728346664360402, -4.548387523817075895 ) ) ;
#12027=EDGE_LOOP ( 'NONE', ( #10132, #4107, #4728, #4846, #3795, #11005 ) ) ;
#12048=CARTESIAN_POINT ( 'NONE',  ( -155.6477983077465410, 110.1970436846185066, 0.000000000000000000 ) ) ;
#12051=CARTESIAN_POINT ( 'NONE',  ( -139.1458939983161827, 103.0129948961282054, 2.431557144026069928 ) ) ;
#12057=ADVANCED_FACE ( 'NONE', ( #1916 ), #10223, .T. ) ;
#12065=DIRECTION ( 'NONE',  ( -0.000000000000000000, -0.000000000000000000, -1.000000000000000000 ) ) ;
#12090=AXIS2_PLACEMENT_3D ( 'NONE', #6122, #7395, #1609 ) ;
#12097=DIRECTION ( 'NONE',  ( -0.4873681696970831312, -0.8731965799097676229, 0.000000000000000000 ) ) ;
#12109=CIRCLE ( 'NONE', #11615, 4.499999999999950262 ) ;
#12135=CARTESIAN_POINT ( 'NONE',  ( -157.6232119703703631, 109.9408540656516067, 9.325089004845752427 ) ) ;
#12179=ORIENTED_EDGE ( 'NONE', *, *, #7021, .F. ) ;
#12182=DIRECTION ( 'NONE',  ( 0.4873681696970824651, 0.8731965799097680669, 0.000000000000000000 ) ) ;
#12184=EDGE_CURVE ( 'NONE', #1565, #2746, #11557, .T. ) ;
#12199=ADVANCED_FACE ( 'NONE', ( #882 ), #8411, .T. ) ;
#12212=CARTESIAN_POINT ( 'NONE',  ( -155.6477983077465410, 110.1970436846185066, 84.88378295107887084 ) ) ;
#12239=AXIS2_PLACEMENT_3D ( 'NONE', #7460, #7390, #6118 ) ;
#12281=DIRECTION ( 'NONE',  ( 0.000000000000000000, 0.000000000000000000, -1.000000000000000000 ) ) ;
#12285=AXIS2_PLACEMENT_3D ( 'NONE', #7911, #3083, #4409 ) ;
#12327=CARTESIAN_POINT ( 'NONE',  ( -151.1649979179899219, 108.2517653509981841, -4.957866620889593179 ) ) ;
#12334=FACE_OUTER_BOUND ( 'NONE', #1086, .T. ) ;
#12337=AXIS2_PLACEMENT_3D ( 'NONE', #4568, #8147, #5681 ) ;
#12340=AXIS2_PLACEMENT_3D ( 'NONE', #981, #15423, #10477 ) ;
#12372=CARTESIAN_POINT ( 'NONE',  ( -151.6951454547776166, 108.2398202450613098, 9.769994122432189343 ) ) ;
#12381=EDGE_CURVE ( 'NONE', #13013, #15505, #13581, .T. ) ;
#12389=DIRECTION ( 'NONE',  ( -0.8731965799097685110, 0.4873681696970816324, 0.000000000000000000 ) ) ;
#12391=EDGE_LOOP ( 'NONE', ( #15231, #13248 ) ) ;
#12393=DIRECTION ( 'NONE',  ( 0.4873681696970815769, 0.8731965799097684000, 0.000000000000000000 ) ) ;
#12414=CARTESIAN_POINT ( 'NONE',  ( -155.8464059187621444, 109.5855229202700087, -4.675203989473057931 ) ) ;
#12419=ADVANCED_FACE ( 'NONE', ( #4921, #3889, #3813 ), #13430, .F. ) ;
#12441=CARTESIAN_POINT ( 'NONE',  ( -157.2827495303359626, 110.9803135124890616, -4.829560219627786921 ) ) ;
#12471=VERTEX_POINT ( 'NONE', #386 ) ;
#12494=ORIENTED_EDGE ( 'NONE', *, *, #8380, .T. ) ;
#12513=CARTESIAN_POINT ( 'NONE',  ( -152.4086188282879277, 107.2728346664360259, 5.000000000000004441 ) ) ;
#12536=PLANE ( 'NONE',  #8812 ) ;
#12549=ORIENTED_EDGE ( 'NONE', *, *, #1025, .T. ) ;
#12595=CARTESIAN_POINT ( 'NONE',  ( -157.6477983077465694, 110.1970436846185208, -4.548387523817069678 ) ) ;
#12601=LINE ( 'NONE', #429, #13571 ) ;
#12606=DIRECTION ( 'NONE',  ( -0.4873681696970814659, -0.8731965799097686221, 0.000000000000000000 ) ) ;
#12665=CARTESIAN_POINT ( 'NONE',  ( -156.6477983077465410, 110.1970436846185066, 0.000000000000000000 ) ) ;
#12680=( NAMED_UNIT ( * ) SI_UNIT ( $, .STERADIAN. ) SOLID_ANGLE_UNIT ( ) );
#12687=DIRECTION ( 'NONE',  ( -1.000000000000000000, 0.000000000000000000, 0.000000000000000000 ) ) ;
#12710=ADVANCED_FACE ( 'NONE', ( #15533, #8396, #13095 ), #11775, .T. ) ;
#12822=DIRECTION ( 'NONE',  ( -1.000000000000000000, 0.000000000000000000, 0.000000000000000000 ) ) ;
#12834=CARTESIAN_POINT ( 'NONE',  ( -152.0432540882499666, 108.0562243547046535, 9.692725945294370149 ) ) ;
#12849=ORIENTED_EDGE ( 'NONE', *, *, #5310, .F. ) ;
#12851=ORIENTED_EDGE ( 'NONE', *, *, #12184, .F. ) ;
#12870=CYLINDRICAL_SURFACE ( 'NONE', #9077, 1.000000000000000888 ) ;
#12896=CONICAL_SURFACE ( 'NONE', #15164, 4.499999999999950262, 0.7853981633974450594 ) ;
#12897=EDGE_CURVE ( 'NONE', #1610, #15505, #6712, .T. ) ;
#12940=VERTEX_POINT ( 'NONE', #8998 ) ;
#12944=ORIENTED_EDGE ( 'NONE', *, *, #14145, .F. ) ;
#12954=CARTESIAN_POINT ( 'NONE',  ( -151.9073788345225466, 106.3957283150743081, 9.183240261263458493 ) ) ;
#12974=CARTESIAN_POINT ( 'NONE',  ( -150.5342426605305945, 106.7706832906523999, -4.718200141660423341 ) ) ;
#12984=CARTESIAN_POINT ( 'NONE',  ( -150.4086188282879277, 107.2728346664360259, 9.719846845941791713 ) ) ;
#12988=VECTOR ( 'NONE', #4035, 999.9999999999998863 ) ;
#13013=VERTEX_POINT ( 'NONE', #4634 ) ;
#13018=VERTEX_POINT ( 'NONE', #3683 ) ;
#13022=VERTEX_POINT ( 'NONE', #41 ) ;
#13036=AXIS2_PLACEMENT_3D ( 'NONE', #1084, #1159, #5988 ) ;
#13056=ORIENTED_EDGE ( 'NONE', *, *, #10337, .F. ) ;
#13095=FACE_OUTER_BOUND ( 'NONE', #4579, .T. ) ;
#13106=PLANE ( 'NONE',  #2802 ) ;
#13157=( LENGTH_UNIT ( ) NAMED_UNIT ( * ) SI_UNIT ( .MILLI., .METRE. ) );
#13228=CARTESIAN_POINT ( 'NONE',  ( -155.7733134923769569, 109.6950568002141324, 9.581378567423390891 ) ) ;
#13241=CARTESIAN_POINT ( 'NONE',  ( -172.4898389879764409, 113.0345383165057314, 2.431557144026070372 ) ) ;
#13247=EDGE_CURVE ( 'NONE', #1565, #6421, #5634, .T. ) ;
#13248=ORIENTED_EDGE ( 'NONE', *, *, #13247, .F. ) ;
#13250=VERTEX_POINT ( 'NONE', #4401 ) ;
#13270=CARTESIAN_POINT ( 'NONE',  ( -150.5371985203381087, 107.7812629986988782, -4.939346198087218198 ) ) ;
#13295=VERTEX_POINT ( 'NONE', #5824 ) ;
#13323=CIRCLE ( 'NONE', #12285, 1.000000000000000888 ) ;
#13338=CARTESIAN_POINT ( 'NONE',  ( -150.4086188282879277, 107.2728346664360259, 9.719846845941791713 ) ) ;
#13398=LINE ( 'NONE', #4000, #6001 ) ;
#13430=PLANE ( 'NONE',  #1655 ) ;
#13436=EDGE_CURVE ( 'NONE', #8424, #14091, #8682, .T. ) ;
#13439=AXIS2_PLACEMENT_3D ( 'NONE', #11438, #2993, #12687 ) ;
#13440=CARTESIAN_POINT ( 'NONE',  ( -157.1441973260925238, 109.3184871819199344, -4.320071790863966754 ) ) ;
#13488=FACE_OUTER_BOUND ( 'NONE', #15569, .T. ) ;
#13501=CARTESIAN_POINT ( 'NONE',  ( -156.4030783857536449, 111.1758453407123852, 9.821053999514624877 ) ) ;
#13544=CARTESIAN_POINT ( 'NONE',  ( -150.4086188282876719, 107.4026543836269525, 9.747367390575380597 ) ) ;
#13554=ORIENTED_EDGE ( 'NONE', *, *, #13247, .T. ) ;
#13571=VECTOR ( 'NONE', #5350, 1000.000000000000227 ) ;
#13573=AXIS2_PLACEMENT_3D ( 'NONE', #3517, #2099, #5968 ) ;
#13581=LINE ( 'NONE', #1351, #12988 ) ;
#13584=DIRECTION ( 'NONE',  ( 0.4873681696970816324, 0.8731965799097685110, -0.000000000000000000 ) ) ;
#13586=ORIENTED_EDGE ( 'NONE', *, *, #9015, .T. ) ;
#13614=DIRECTION ( 'NONE',  ( -0.4873681696970831312, -0.8731965799097676229, 0.000000000000000000 ) ) ;
#13660=CARTESIAN_POINT ( 'NONE',  ( -157.6477983077465694, 110.1970436846184924, 9.411501811869198875 ) ) ;
#13672=CARTESIAN_POINT ( 'NONE',  ( -157.6477983077465694, 110.1970436846185208, -4.548387523817069678 ) ) ;
#13680=CARTESIAN_POINT ( 'NONE',  ( -139.1458939983161827, 103.0129948961282054, 2.431557144026069928 ) ) ;
#13703=CARTESIAN_POINT ( 'NONE',  ( -157.6240445055952648, 110.4483201618638191, -4.636096941365077662 ) ) ;
#13738=CARTESIAN_POINT ( 'NONE',  ( -156.8030008057995985, 111.1938936318135376, 9.788006227097792333 ) ) ;
#13776=VECTOR ( 'NONE', #2440, 1000.000000000000114 ) ;
#13805=CARTESIAN_POINT ( 'NONE',  ( -139.1458939983161827, 103.0129948961282054, 5.000000000000000000 ) ) ;
#13876=VECTOR ( 'NONE', #2586, 1000.000000000000000 ) ;
#13883=VECTOR ( 'NONE', #8487, 999.9999999999998863 ) ;
#13888=EDGE_LOOP ( 'NONE', ( #5918, #8419, #11000, #14534 ) ) ;
#13899=SHAPE_DEFINITION_REPRESENTATION ( #9550, #10258 ) ;
#13903=ORIENTED_EDGE ( 'NONE', *, *, #13436, .F. ) ;
#13915=CYLINDRICAL_SURFACE ( 'NONE', #750, 7.499999999999999112 ) ;
#13923=ADVANCED_FACE ( 'NONE', ( #7847 ), #9021, .F. ) ;
#13950=CARTESIAN_POINT ( 'NONE',  ( -152.4086188282879561, 107.4000165207912261, 9.455162786586091883 ) ) ;
#13980=EDGE_LOOP ( 'NONE', ( #2104, #13586 ) ) ;
#13990=DIRECTION ( 'NONE',  ( -0.4873681696970814659, -0.8731965799097686221, 0.000000000000000000 ) ) ;
#14018=EDGE_CURVE ( 'NONE', #9103, #5262, #11696, .T. ) ;
#14026=DIRECTION ( 'NONE',  ( -0.8731965799097684000, 0.4873681696970815769, 0.000000000000000000 ) ) ;
#14038=CARTESIAN_POINT ( 'NONE',  ( -150.4086188282879277, 107.2728346664360259, 84.88378295107887084 ) ) ;
#14060=DIRECTION ( 'NONE',  ( -0.4873681696970814659, -0.8731965799097686221, 0.000000000000000000 ) ) ;
#14091=VERTEX_POINT ( 'NONE', #2353 ) ;
#14145=EDGE_CURVE ( 'NONE', #13250, #6618, #5242, .T. ) ;
#14151=CARTESIAN_POINT ( 'NONE',  ( -215.1139964504661464, 145.4140256597743814, 2.431557144026069928 ) ) ;
#14217=VECTOR ( 'NONE', #12393, 1000.000000000000114 ) ;
#14238=AXIS2_PLACEMENT_3D ( 'NONE', #11719, #4440, #9273 ) ;
#14250=ORIENTED_EDGE ( 'NONE', *, *, #15246, .T. ) ;
#14256=DIRECTION ( 'NONE',  ( 0.000000000000000000, -0.000000000000000000, -1.000000000000000000 ) ) ;
#14257=DIRECTION ( 'NONE',  ( -0.8731965799097685110, 0.4873681696970816324, 0.000000000000000000 ) ) ;
#14290=CARTESIAN_POINT ( 'NONE',  ( -151.1267316678846839, 106.2776699442079433, 9.312033302791153488 ) ) ;
#14307=CARTESIAN_POINT ( 'NONE',  ( -151.4086188282879277, 107.2728346664360259, 84.88378295107887084 ) ) ;
#14369=CARTESIAN_POINT ( 'NONE',  ( -170.8906599468338641, 95.38134948400895041, 0.000000000000000000 ) ) ;
#14378=CARTESIAN_POINT ( 'NONE',  ( -222.0995690897442785, 149.3129710173510318, 2.431557144026069928 ) ) ;
#14379=AXIS2_PLACEMENT_3D ( 'NONE', #6546, #9940, #14799 ) ;
#14497=( NAMED_UNIT ( * ) PLANE_ANGLE_UNIT ( ) SI_UNIT ( $, .RADIAN. ) );
#14518=EDGE_CURVE ( 'NONE', #6255, #12471, #7293, .T. ) ;
#14533=CARTESIAN_POINT ( 'NONE',  ( -151.5642236857922001, 108.2694729682366841, -4.924812526309171545 ) ) ;
#14534=ORIENTED_EDGE ( 'NONE', *, *, #8380, .F. ) ;
#14577=DIRECTION ( 'NONE',  ( 0.8731965799097685110, -0.4873681696970816879, -0.000000000000000000 ) ) ;
#14615=AXIS2_PLACEMENT_3D ( 'NONE', #5706, #5629, #14060 ) ;
#14623=CARTESIAN_POINT ( 'NONE',  ( -157.6477983077465694, 110.1970436846185066, 0.000000000000000000 ) ) ;
#14627=ADVANCED_FACE ( 'NONE', ( #2014 ), #1142, .F. ) ;
#14646=CARTESIAN_POINT ( 'NONE',  ( -150.4086188282879277, 107.2728346664360259, -4.856732557889654522 ) ) ;
#14661=CARTESIAN_POINT ( 'NONE',  ( -224.2927258533811425, 145.3835864077571216, 2.431557144026069928 ) ) ;
#14691=CARTESIAN_POINT ( 'NONE',  ( -152.2217123724471435, 107.8691177927835838, -4.760088435541713459 ) ) ;
#14712=VERTEX_POINT ( 'NONE', #12984 ) ;
#14725=ADVANCED_FACE ( 'NONE', ( #2726 ), #11101, .F. ) ;
#14729=DIRECTION ( 'NONE',  ( 0.000000000000000000, 0.000000000000000000, -1.000000000000000000 ) ) ;
#14734=CARTESIAN_POINT ( 'NONE',  ( -151.2970693524540877, 108.2755082659018768, 9.813568765712858522 ) ) ;
#14763=CARTESIAN_POINT ( 'NONE',  ( -156.5362488319127579, 111.1997172840843575, 9.813568765712854969 ) ) ;
#14767=DIRECTION ( 'NONE',  ( -0.8731965799097685110, 0.4873681696970816324, 0.000000000000000000 ) ) ;
#14778=ORIENTED_EDGE ( 'NONE', *, *, #1850, .F. ) ;
#14782=ORIENTED_EDGE ( 'NONE', *, *, #5603, .F. ) ;
#14795=APPLICATION_CONTEXT ( 'automotive_design' ) ;
#14799=DIRECTION ( 'NONE',  ( -1.000000000000000000, 0.000000000000000000, -0.000000000000000000 ) ) ;
#14820=ORIENTED_EDGE ( 'NONE', *, *, #4078, .F. ) ;
#14826=LINE ( 'NONE', #7838, #5378 ) ;
#14836=CARTESIAN_POINT ( 'NONE',  ( -157.6477983077465979, 110.3242255389737068, 9.455162786586084778 ) ) ;
#14852=CARTESIAN_POINT ( 'NONE',  ( -156.8931177578041343, 109.2182220046010173, -4.336802791931503087 ) ) ;
#14910=LINE ( 'NONE', #13805, #14217 ) ;
#14948=DIRECTION ( 'NONE',  ( -1.000000000000000000, 0.000000000000000000, 0.000000000000000000 ) ) ;
#14957=CARTESIAN_POINT ( 'NONE',  ( -157.6477983077465410, 110.3243625741235974, -4.592095542101950478 ) ) ;
#14995=CARTESIAN_POINT ( 'NONE',  ( -156.9343249342362583, 111.1640292632437905, 9.769994122432187567 ) ) ;
#15005=EDGE_LOOP ( 'NONE', ( #4900, #11854 ) ) ;
#15020=EDGE_LOOP ( 'NONE', ( #1588, #15564 ) ) ;
#15034=CARTESIAN_POINT ( 'NONE',  ( -156.0423532639127018, 111.0040250659683068, -4.962432776364138043 ) ) ;
#15136=ORIENTED_EDGE ( 'NONE', *, *, #11927, .F. ) ;
#15164=AXIS2_PLACEMENT_3D ( 'NONE', #10314, #5336, #11572 ) ;
#15190=DIRECTION ( 'NONE',  ( -0.4873681696970831312, -0.8731965799097676229, 0.000000000000000000 ) ) ;
#15231=ORIENTED_EDGE ( 'NONE', *, *, #10642, .F. ) ;
#15242=AXIS2_PLACEMENT_3D ( 'NONE', #14378, #9660, #5713 ) ;
#15246=EDGE_CURVE ( 'NONE', #14091, #8424, #9324, .T. ) ;
#15260=ORIENTED_EDGE ( 'NONE', *, *, #4301, .T. ) ;
#15273=EDGE_CURVE ( 'NONE', #6329, #3093, #10539, .T. ) ;
#15305=ORIENTED_EDGE ( 'NONE', *, *, #2284, .F. ) ;
#15364=LINE ( 'NONE', #3855, #3573 ) ;
#15367=VECTOR ( 'NONE', #10800, 999.9999999999998863 ) ;
#15374=VECTOR ( 'NONE', #4488, 999.9999999999998863 ) ;
#15408=ADVANCED_FACE ( 'NONE', ( #4263 ), #3959, .F. ) ;
#15414=CARTESIAN_POINT ( 'NONE',  ( -151.5195349256774762, 106.2703939966685027, -4.358407942927359002 ) ) ;
#15423=DIRECTION ( 'NONE',  ( 0.000000000000000000, 0.000000000000000000, -1.000000000000000000 ) ) ;
#15472=FACE_BOUND ( 'NONE', #6351, .T. ) ;
#15491=CYLINDRICAL_SURFACE ( 'NONE', #7058, 1.000000000000000888 ) ;
#15505=VERTEX_POINT ( 'NONE', #8003 ) ;
#15521=EDGE_LOOP ( 'NONE', ( #2933, #2564 ) ) ;
#15523=LINE ( 'NONE', #4808, #8552 ) ;
#15529=ORIENTED_EDGE ( 'NONE', *, *, #7018, .F. ) ;
#15533=FACE_BOUND ( 'NONE', #8078, .T. ) ;
#15550=ADVANCED_FACE ( 'NONE', ( #10512 ), #12870, .F. ) ;
#15561=CYLINDRICAL_SURFACE ( 'NONE', #6974, 1.000000000000000888 ) ;
#15564=ORIENTED_EDGE ( 'NONE', *, *, #8384, .F. ) ;
#15569=EDGE_LOOP ( 'NONE', ( #8830, #1177, #4842, #2536, #3156 ) ) ;
#15589=LINE ( 'NONE', #39, #13876 ) ;
ENDSEC;
END-ISO-10303-21;
